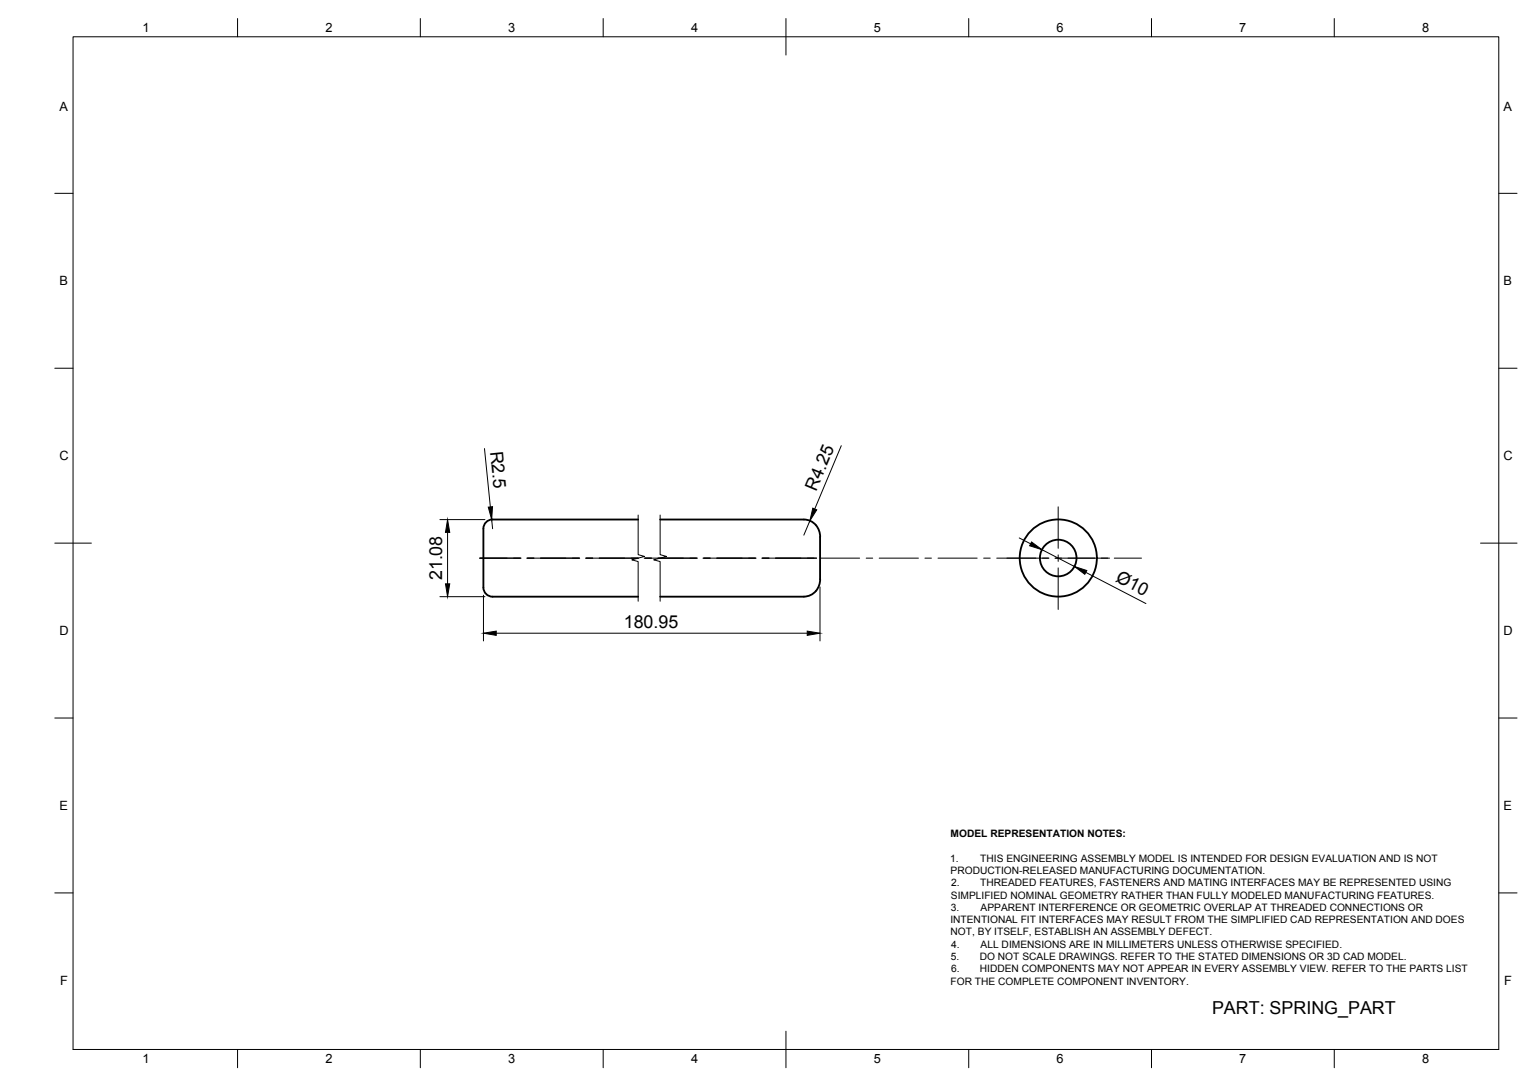
ISO-10303-21;
HEADER;
/* Generated by software containing ST-Developer
 * from STEP Tools, Inc. (www.steptools.com) 
 */

FILE_DESCRIPTION(
/* description */ (''),
/* implementation_level */ '2;1');

FILE_NAME(
/* name */ 'Spring_part.step',
/* time_stamp */ '2026-10-04T16:49:01-07:00',
/* author */ (''),
/* organization */ (''),
/* preprocessor_version */ 'ST-DEVELOPER v20.2',
/* originating_system */ 'Autodesk Translation Framework v15.15.0.0',
/* authorisation */ '');

FILE_SCHEMA (('AUTOMOTIVE_DESIGN { 1 0 10303 214 3 1 1 }'));
ENDSEC;

DATA;
#10=MECHANICAL_DESIGN_GEOMETRIC_PRESENTATION_REPRESENTATION('',(#83),#51553);
#45=TOROIDAL_SURFACE('',#4496,8.03882147643231,2.49999999999996);
#46=TOROIDAL_SURFACE('',#4502,5.78096926885271,5.05765846207533);
#47=TOROIDAL_SURFACE('',#4505,6.2888214764323,4.24999999999998);
#67=SHAPE_REPRESENTATION_RELATIONSHIP('SRR','None',#51588,#75);
#75=ADVANCED_BREP_SHAPE_REPRESENTATION('',(#92),#51548);
#83=STYLED_ITEM('',(#51635),#92);
#92=MANIFOLD_SOLID_BREP('Body1',#4262);
#106=FACE_BOUND('',#482,.T.);
#107=FACE_BOUND('',#484,.T.);
#147=PLANE('',#4499);
#148=PLANE('',#4500);
#275=FACE_OUTER_BOUND('',#478,.T.);
#276=FACE_OUTER_BOUND('',#479,.T.);
#277=FACE_OUTER_BOUND('',#480,.T.);
#278=FACE_OUTER_BOUND('',#481,.T.);
#279=FACE_OUTER_BOUND('',#483,.T.);
#280=FACE_OUTER_BOUND('',#485,.T.);
#281=FACE_OUTER_BOUND('',#486,.T.);
#478=EDGE_LOOP('',(#3273,#3274,#3275,#3276));
#479=EDGE_LOOP('',(#3277,#3278,#3279,#3280));
#480=EDGE_LOOP('',(#3281,#3282,#3283,#3284));
#481=EDGE_LOOP('',(#3285));
#482=EDGE_LOOP('',(#3286));
#483=EDGE_LOOP('',(#3287));
#484=EDGE_LOOP('',(#3288));
#485=EDGE_LOOP('',(#3289,#3290,#3291,#3292));
#486=EDGE_LOOP('',(#3293,#3294,#3295,#3296));
#639=CIRCLE('',#4491,5.);
#640=CIRCLE('',#4492,5.);
#641=CIRCLE('',#4494,10.5388214764323);
#642=CIRCLE('',#4495,10.5388214764323);
#643=CIRCLE('',#4497,8.03882147643229);
#644=CIRCLE('',#4498,2.49999999999996);
#645=CIRCLE('',#4501,5.78096926885272);
#646=CIRCLE('',#4503,8.96120340959139);
#647=CIRCLE('',#4504,5.05765846207533);
#648=CIRCLE('',#4506,4.24999999999998);
#824=LINE('',#28089,#1052);
#825=LINE('',#28095,#1053);
#1052=VECTOR('',#5054,5.);
#1053=VECTOR('',#5061,10.5388214764323);
#1716=VERTEX_POINT('',#28086);
#1717=VERTEX_POINT('',#28088);
#1718=VERTEX_POINT('',#28092);
#1719=VERTEX_POINT('',#28094);
#1720=VERTEX_POINT('',#28098);
#1721=VERTEX_POINT('',#28103);
#1722=VERTEX_POINT('',#28106);
#2290=EDGE_CURVE('',#1716,#1716,#639,.T.);
#2291=EDGE_CURVE('',#1716,#1717,#824,.T.);
#2292=EDGE_CURVE('',#1717,#1717,#640,.T.);
#2293=EDGE_CURVE('',#1718,#1718,#641,.T.);
#2294=EDGE_CURVE('',#1718,#1719,#825,.T.);
#2295=EDGE_CURVE('',#1719,#1719,#642,.T.);
#2296=EDGE_CURVE('',#1720,#1720,#643,.T.);
#2297=EDGE_CURVE('',#1720,#1718,#644,.T.);
#2298=EDGE_CURVE('',#1721,#1721,#645,.T.);
#2299=EDGE_CURVE('',#1722,#1722,#646,.T.);
#2300=EDGE_CURVE('',#1722,#1721,#647,.T.);
#2301=EDGE_CURVE('',#1719,#1722,#648,.T.);
#3273=ORIENTED_EDGE('',*,*,#2290,.F.);
#3274=ORIENTED_EDGE('',*,*,#2291,.T.);
#3275=ORIENTED_EDGE('',*,*,#2292,.F.);
#3276=ORIENTED_EDGE('',*,*,#2291,.F.);
#3277=ORIENTED_EDGE('',*,*,#2293,.F.);
#3278=ORIENTED_EDGE('',*,*,#2294,.T.);
#3279=ORIENTED_EDGE('',*,*,#2295,.T.);
#3280=ORIENTED_EDGE('',*,*,#2294,.F.);
#3281=ORIENTED_EDGE('',*,*,#2296,.F.);
#3282=ORIENTED_EDGE('',*,*,#2297,.T.);
#3283=ORIENTED_EDGE('',*,*,#2293,.T.);
#3284=ORIENTED_EDGE('',*,*,#2297,.F.);
#3285=ORIENTED_EDGE('',*,*,#2296,.T.);
#3286=ORIENTED_EDGE('',*,*,#2290,.T.);
#3287=ORIENTED_EDGE('',*,*,#2298,.F.);
#3288=ORIENTED_EDGE('',*,*,#2292,.T.);
#3289=ORIENTED_EDGE('',*,*,#2299,.F.);
#3290=ORIENTED_EDGE('',*,*,#2300,.T.);
#3291=ORIENTED_EDGE('',*,*,#2298,.T.);
#3292=ORIENTED_EDGE('',*,*,#2300,.F.);
#3293=ORIENTED_EDGE('',*,*,#2295,.F.);
#3294=ORIENTED_EDGE('',*,*,#2301,.T.);
#3295=ORIENTED_EDGE('',*,*,#2299,.T.);
#3296=ORIENTED_EDGE('',*,*,#2301,.F.);
#4006=CYLINDRICAL_SURFACE('',#4490,5.);
#4007=CYLINDRICAL_SURFACE('',#4493,10.5388214764323);
#4158=ADVANCED_FACE('',(#275),#4006,.F.);
#4159=ADVANCED_FACE('',(#276),#4007,.T.);
#4160=ADVANCED_FACE('',(#277),#45,.T.);
#4161=ADVANCED_FACE('',(#278,#106),#147,.T.);
#4162=ADVANCED_FACE('',(#279,#107),#148,.T.);
#4163=ADVANCED_FACE('',(#280),#46,.T.);
#4164=ADVANCED_FACE('',(#281),#47,.T.);
#4262=CLOSED_SHELL('',(#4158,#4159,#4160,#4161,#4162,#4163,#4164));
#4489=AXIS2_PLACEMENT_3D('',#28084,#5048,#5049);
#4490=AXIS2_PLACEMENT_3D('',#28085,#5050,#5051);
#4491=AXIS2_PLACEMENT_3D('',#28087,#5052,#5053);
#4492=AXIS2_PLACEMENT_3D('',#28090,#5055,#5056);
#4493=AXIS2_PLACEMENT_3D('',#28091,#5057,#5058);
#4494=AXIS2_PLACEMENT_3D('',#28093,#5059,#5060);
#4495=AXIS2_PLACEMENT_3D('',#28096,#5062,#5063);
#4496=AXIS2_PLACEMENT_3D('',#28097,#5064,#5065);
#4497=AXIS2_PLACEMENT_3D('',#28099,#5066,#5067);
#4498=AXIS2_PLACEMENT_3D('',#28100,#5068,#5069);
#4499=AXIS2_PLACEMENT_3D('',#28101,#5070,#5071);
#4500=AXIS2_PLACEMENT_3D('',#28102,#5072,#5073);
#4501=AXIS2_PLACEMENT_3D('',#28104,#5074,#5075);
#4502=AXIS2_PLACEMENT_3D('',#28105,#5076,#5077);
#4503=AXIS2_PLACEMENT_3D('',#28107,#5078,#5079);
#4504=AXIS2_PLACEMENT_3D('',#28108,#5080,#5081);
#4505=AXIS2_PLACEMENT_3D('',#28109,#5082,#5083);
#4506=AXIS2_PLACEMENT_3D('',#28110,#5084,#5085);
#5048=DIRECTION('axis',(0.,0.,1.));
#5049=DIRECTION('refdir',(1.,0.,0.));
#5050=DIRECTION('center_axis',(-1.,0.,0.));
#5051=DIRECTION('ref_axis',(0.,1.,0.));
#5052=DIRECTION('center_axis',(-1.,0.,0.));
#5053=DIRECTION('ref_axis',(0.,1.,0.));
#5054=DIRECTION('',(-1.,0.,0.));
#5055=DIRECTION('center_axis',(1.,0.,0.));
#5056=DIRECTION('ref_axis',(0.,1.,0.));
#5057=DIRECTION('center_axis',(1.,0.,0.));
#5058=DIRECTION('ref_axis',(0.,0.,-1.));
#5059=DIRECTION('center_axis',(1.,0.,0.));
#5060=DIRECTION('ref_axis',(0.,0.,-1.));
#5061=DIRECTION('',(-1.,0.,0.));
#5062=DIRECTION('center_axis',(1.,0.,0.));
#5063=DIRECTION('ref_axis',(0.,0.,-1.));
#5064=DIRECTION('center_axis',(1.,0.,0.));
#5065=DIRECTION('ref_axis',(0.,0.,-1.));
#5066=DIRECTION('center_axis',(1.,0.,0.));
#5067=DIRECTION('ref_axis',(0.,0.,-1.));
#5068=DIRECTION('center_axis',(0.,-1.,-1.22464679914735E-16));
#5069=DIRECTION('ref_axis',(0.,-1.22464679914735E-16,1.));
#5070=DIRECTION('center_axis',(1.,0.,0.));
#5071=DIRECTION('ref_axis',(0.,0.,-1.));
#5072=DIRECTION('center_axis',(-1.,0.,0.));
#5073=DIRECTION('ref_axis',(0.,0.,1.));
#5074=DIRECTION('center_axis',(1.,0.,0.));
#5075=DIRECTION('ref_axis',(0.,0.,-1.));
#5076=DIRECTION('center_axis',(1.,0.,0.));
#5077=DIRECTION('ref_axis',(0.,0.,-1.));
#5078=DIRECTION('center_axis',(1.,0.,0.));
#5079=DIRECTION('ref_axis',(0.,0.,-1.));
#5080=DIRECTION('center_axis',(0.,-1.,-1.22464679914735E-16));
#5081=DIRECTION('ref_axis',(0.,-1.22464679914735E-16,1.));
#5082=DIRECTION('center_axis',(1.,0.,0.));
#5083=DIRECTION('ref_axis',(0.,0.,-1.));
#5084=DIRECTION('center_axis',(0.,-1.,-1.22464679914735E-16));
#5085=DIRECTION('ref_axis',(0.,-1.22464679914735E-16,1.));
#28084=CARTESIAN_POINT('',(0.,0.,0.));
#28085=CARTESIAN_POINT('Origin',(206.833344075386,0.,0.));
#28086=CARTESIAN_POINT('',(206.833344075386,-5.,-6.12323399573677E-16));
#28087=CARTESIAN_POINT('Origin',(206.833344075386,0.,0.));
#28088=CARTESIAN_POINT('',(25.8804751042881,-5.,-6.12323399573677E-16));
#28089=CARTESIAN_POINT('',(206.833344075386,-5.,6.12323399573677E-16));
#28090=CARTESIAN_POINT('Origin',(25.8804751042881,0.,0.));
#28091=CARTESIAN_POINT('Origin',(117.321733117655,0.,0.));
#28092=CARTESIAN_POINT('',(204.333344075386,-1.29063339878982E-15,10.5388214764323));
#28093=CARTESIAN_POINT('Origin',(204.333344075386,0.,0.));
#28094=CARTESIAN_POINT('',(30.3101221599236,-1.29063339878982E-15,10.5388214764323));
#28095=CARTESIAN_POINT('',(117.321733117655,-1.29063339878982E-15,10.5388214764323));
#28096=CARTESIAN_POINT('Origin',(30.3101221599236,0.,0.));
#28097=CARTESIAN_POINT('Origin',(204.333344075386,0.,0.));
#28098=CARTESIAN_POINT('',(206.833344075386,-9.8447169900298E-16,8.03882147643229));
#28099=CARTESIAN_POINT('Origin',(206.833344075386,0.,0.));
#28100=CARTESIAN_POINT('Origin',(204.333344075386,-9.84471699002983E-16,
8.03882147643231));
#28101=CARTESIAN_POINT('Origin',(206.833344075386,0.,0.));
#28102=CARTESIAN_POINT('Origin',(25.8804751042881,0.,-5.78096926885272));
#28103=CARTESIAN_POINT('',(25.8804751042881,-7.0796455110697E-16,5.78096926885272));
#28104=CARTESIAN_POINT('Origin',(25.8804751042881,0.,0.));
#28105=CARTESIAN_POINT('Origin',(30.9381335663634,0.,0.));
#28106=CARTESIAN_POINT('',(27.0054474704383,-1.09743090720644E-15,8.96120340959139));
#28107=CARTESIAN_POINT('Origin',(27.0054474704383,0.,0.));
#28108=CARTESIAN_POINT('Origin',(30.9381335663634,-7.07964551106969E-16,
5.78096926885271));
#28109=CARTESIAN_POINT('Origin',(30.3101221599236,0.,0.));
#28110=CARTESIAN_POINT('Origin',(30.3101221599236,-7.70158509152195E-16,
6.2888214764323));
#51538=UNCERTAINTY_MEASURE_WITH_UNIT(LENGTH_MEASURE(0.01),#51554,
'DISTANCE_ACCURACY_VALUE',
'Maximum model space distance between geometric entities at asserted c
onnectivities');
#51543=UNCERTAINTY_MEASURE_WITH_UNIT(LENGTH_MEASURE(0.01),#51554,
'DISTANCE_ACCURACY_VALUE',
'Maximum model space distance between geometric entities at asserted c
onnectivities');
#51548=(
GEOMETRIC_REPRESENTATION_CONTEXT(3)
GLOBAL_UNCERTAINTY_ASSIGNED_CONTEXT((#51538))
GLOBAL_UNIT_ASSIGNED_CONTEXT((#51554,#51556,#51557))
REPRESENTATION_CONTEXT('','3D')
);
#51553=(
GEOMETRIC_REPRESENTATION_CONTEXT(3)
GLOBAL_UNCERTAINTY_ASSIGNED_CONTEXT((#51543))
GLOBAL_UNIT_ASSIGNED_CONTEXT((#51554,#51556,#51557))
REPRESENTATION_CONTEXT('','3D')
);
#51554=(
LENGTH_UNIT()
NAMED_UNIT(*)
SI_UNIT(.MILLI.,.METRE.)
);
#51556=(
NAMED_UNIT(*)
PLANE_ANGLE_UNIT()
SI_UNIT($,.RADIAN.)
);
#51557=(
NAMED_UNIT(*)
SI_UNIT($,.STERADIAN.)
SOLID_ANGLE_UNIT()
);
#51562=SHAPE_DEFINITION_REPRESENTATION(#51571,#51588);
#51571=PRODUCT_DEFINITION_SHAPE('',$,#51598);
#51588=SHAPE_REPRESENTATION('',(#4489),#51548);
#51593=PRODUCT_DEFINITION_CONTEXT('part definition',#51622,'design');
#51598=PRODUCT_DEFINITION('Spring_part','Spring_part',#51607,#51593);
#51607=PRODUCT_DEFINITION_FORMATION('',$,#51628);
#51622=APPLICATION_CONTEXT(
'Core Data for Automotive Mechanical Design Process');
#51623=PRODUCT_CONTEXT('part definition',#51622,'mechanical');
#51628=PRODUCT('Spring_part','Spring_part',$,(#51623));
#51635=PRESENTATION_STYLE_ASSIGNMENT((#51638));
#51638=SURFACE_STYLE_USAGE(.BOTH.,#51641);
#51641=SURFACE_SIDE_STYLE('',(#51644));
#51644=SURFACE_STYLE_FILL_AREA(#51647);
#51647=FILL_AREA_STYLE('Opaque(60,60,60)',(#51650));
#51650=FILL_AREA_STYLE_COLOUR('Opaque(60,60,60)',#51653);
#51653=COLOUR_RGB('Opaque(60,60,60)', 0.40784314, 0.44705882, 0.49803922);
ENDSEC;
END-ISO-10303-21;
